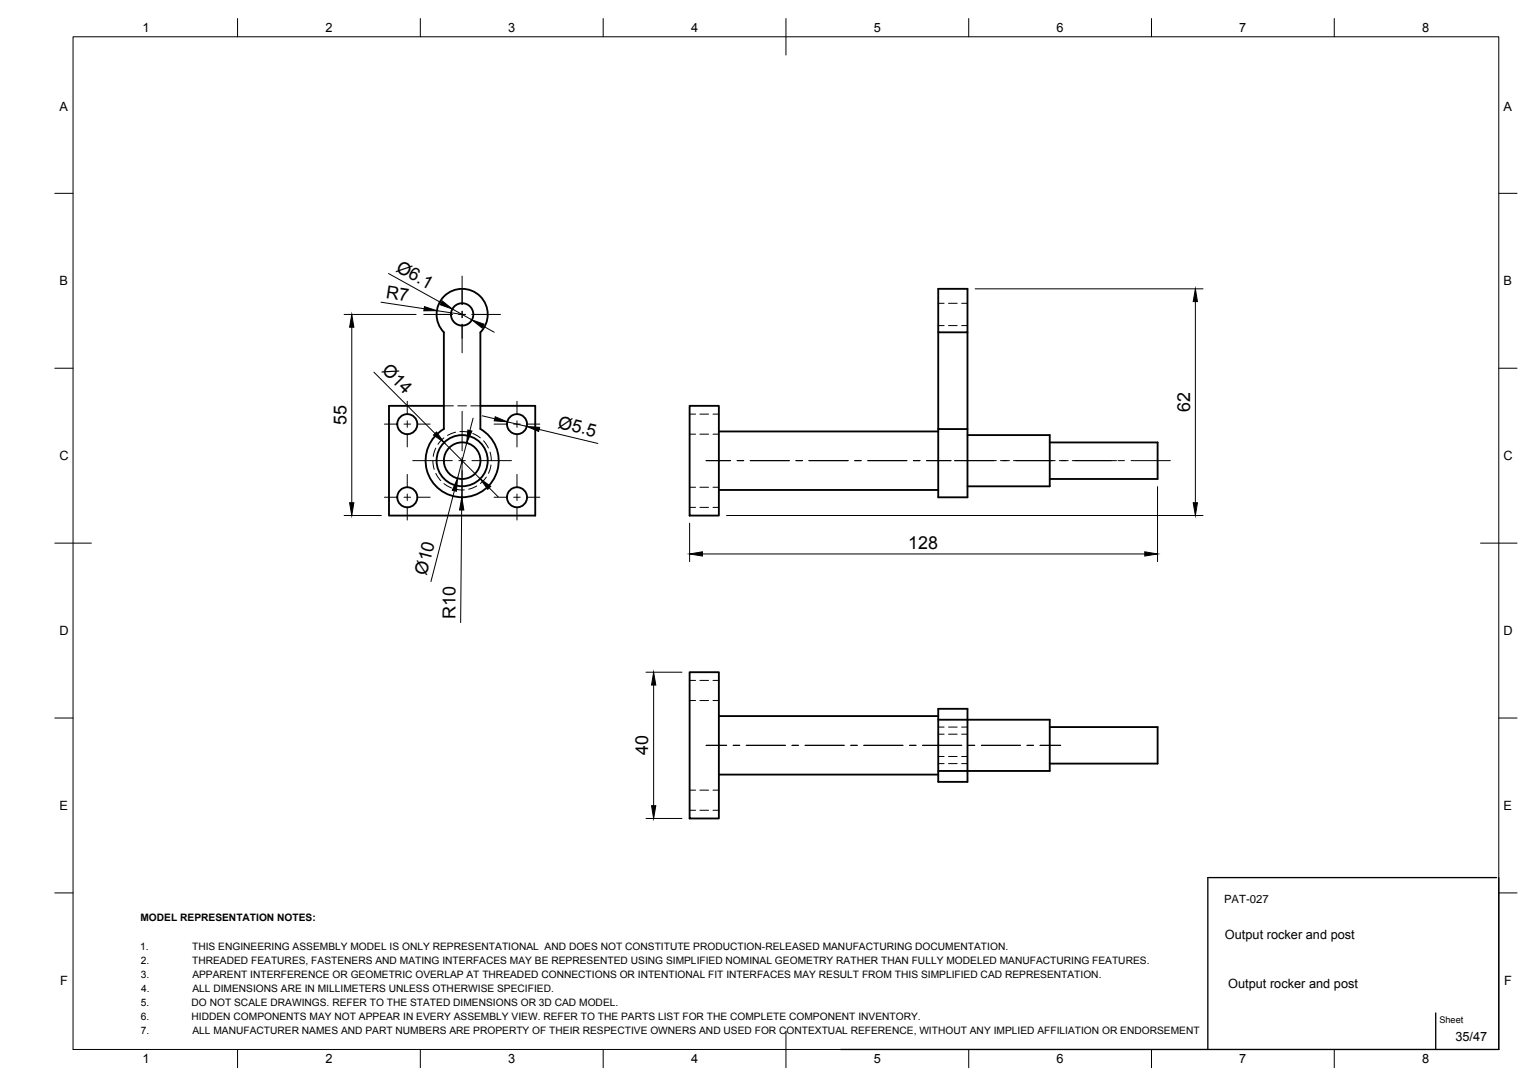
ISO-10303-21;
HEADER;
/* Generated by software containing ST-Developer
 * from STEP Tools, Inc. (www.steptools.com) 
 */

FILE_DESCRIPTION(
/* description */ ('Crank-driven oscillating fan base (mechanism only)'),

/* implementation_level */ '2;1');

FILE_NAME(
/* name */ 'Output rocker and post.step',
/* time_stamp */ '2026-10-28T03:25:00-07:00',
/* author */ (''),
/* organization */ (''),
/* preprocessor_version */ 'ST-DEVELOPER v20.2',
/* originating_system */ 'Autodesk Translation Framework v15.17.0.0',
/* authorisation */ '');

FILE_SCHEMA (('AUTOMOTIVE_DESIGN { 1 0 10303 214 3 1 1 }'));
ENDSEC;

DATA;
#10=MECHANICAL_DESIGN_GEOMETRIC_PRESENTATION_REPRESENTATION('',(#471),#11916);
#383=SHAPE_REPRESENTATION_RELATIONSHIP('SRR','None',#12110,#423);
#423=ADVANCED_BREP_SHAPE_REPRESENTATION('',(#518),#11901);
#471=STYLED_ITEM('',(#12361),#518);
#518=MANIFOLD_SOLID_BREP('Body1',#6102);
#649=FACE_BOUND('',#1640,.T.);
#650=FACE_BOUND('',#1641,.T.);
#651=FACE_BOUND('',#1642,.T.);
#652=FACE_BOUND('',#1643,.T.);
#653=FACE_BOUND('',#1644,.T.);
#654=FACE_BOUND('',#1650,.T.);
#655=FACE_BOUND('',#1651,.T.);
#656=FACE_BOUND('',#1652,.T.);
#657=FACE_BOUND('',#1653,.T.);
#658=FACE_BOUND('',#1659,.T.);
#659=FACE_BOUND('',#1660,.T.);
#660=FACE_BOUND('',#1664,.T.);
#661=FACE_BOUND('',#1665,.T.);
#662=FACE_BOUND('',#1667,.T.);
#815=PLANE('',#7138);
#816=PLANE('',#7140);
#817=PLANE('',#7141);
#818=PLANE('',#7142);
#819=PLANE('',#7143);
#820=PLANE('',#7144);
#821=PLANE('',#7153);
#822=PLANE('',#7154);
#823=PLANE('',#7156);
#824=PLANE('',#7159);
#825=PLANE('',#7161);
#826=PLANE('',#7167);
#1141=FACE_OUTER_BOUND('',#1635,.T.);
#1142=FACE_OUTER_BOUND('',#1636,.T.);
#1143=FACE_OUTER_BOUND('',#1637,.T.);
#1144=FACE_OUTER_BOUND('',#1638,.T.);
#1145=FACE_OUTER_BOUND('',#1639,.T.);
#1146=FACE_OUTER_BOUND('',#1645,.T.);
#1147=FACE_OUTER_BOUND('',#1646,.T.);
#1148=FACE_OUTER_BOUND('',#1647,.T.);
#1149=FACE_OUTER_BOUND('',#1648,.T.);
#1150=FACE_OUTER_BOUND('',#1649,.T.);
#1151=FACE_OUTER_BOUND('',#1654,.T.);
#1152=FACE_OUTER_BOUND('',#1655,.T.);
#1153=FACE_OUTER_BOUND('',#1656,.T.);
#1154=FACE_OUTER_BOUND('',#1657,.T.);
#1155=FACE_OUTER_BOUND('',#1658,.T.);
#1156=FACE_OUTER_BOUND('',#1661,.T.);
#1157=FACE_OUTER_BOUND('',#1662,.T.);
#1158=FACE_OUTER_BOUND('',#1663,.T.);
#1159=FACE_OUTER_BOUND('',#1666,.T.);
#1160=FACE_OUTER_BOUND('',#1668,.T.);
#1161=FACE_OUTER_BOUND('',#1669,.T.);
#1162=FACE_OUTER_BOUND('',#1670,.T.);
#1635=EDGE_LOOP('',(#5098,#5099,#5100,#5101));
#1636=EDGE_LOOP('',(#5102,#5103,#5104,#5105));
#1637=EDGE_LOOP('',(#5106,#5107,#5108,#5109));
#1638=EDGE_LOOP('',(#5110,#5111,#5112,#5113));
#1639=EDGE_LOOP('',(#5114,#5115,#5116,#5117));
#1640=EDGE_LOOP('',(#5118));
#1641=EDGE_LOOP('',(#5119));
#1642=EDGE_LOOP('',(#5120));
#1643=EDGE_LOOP('',(#5121));
#1644=EDGE_LOOP('',(#5122));
#1645=EDGE_LOOP('',(#5123,#5124,#5125,#5126));
#1646=EDGE_LOOP('',(#5127,#5128,#5129,#5130));
#1647=EDGE_LOOP('',(#5131,#5132,#5133,#5134));
#1648=EDGE_LOOP('',(#5135,#5136,#5137,#5138));
#1649=EDGE_LOOP('',(#5139,#5140,#5141,#5142));
#1650=EDGE_LOOP('',(#5143));
#1651=EDGE_LOOP('',(#5144));
#1652=EDGE_LOOP('',(#5145));
#1653=EDGE_LOOP('',(#5146));
#1654=EDGE_LOOP('',(#5147,#5148,#5149,#5150));
#1655=EDGE_LOOP('',(#5151,#5152,#5153,#5154));
#1656=EDGE_LOOP('',(#5155,#5156,#5157,#5158));
#1657=EDGE_LOOP('',(#5159,#5160,#5161,#5162));
#1658=EDGE_LOOP('',(#5163,#5164,#5165,#5166));
#1659=EDGE_LOOP('',(#5167));
#1660=EDGE_LOOP('',(#5168));
#1661=EDGE_LOOP('',(#5169,#5170,#5171,#5172));
#1662=EDGE_LOOP('',(#5173,#5174,#5175,#5176));
#1663=EDGE_LOOP('',(#5177,#5178,#5179,#5180));
#1664=EDGE_LOOP('',(#5181));
#1665=EDGE_LOOP('',(#5182));
#1666=EDGE_LOOP('',(#5183));
#1667=EDGE_LOOP('',(#5184));
#1668=EDGE_LOOP('',(#5185,#5186,#5187,#5188));
#1669=EDGE_LOOP('',(#5189,#5190,#5191,#5192));
#1670=EDGE_LOOP('',(#5193));
#2002=LINE('',#11200,#2335);
#2003=LINE('',#11206,#2336);
#2004=LINE('',#11212,#2337);
#2005=LINE('',#11218,#2338);
#2006=LINE('',#11223,#2339);
#2007=LINE('',#11225,#2340);
#2008=LINE('',#11227,#2341);
#2009=LINE('',#11228,#2342);
#2010=LINE('',#11233,#2343);
#2011=LINE('',#11235,#2344);
#2012=LINE('',#11236,#2345);
#2013=LINE('',#11239,#2346);
#2014=LINE('',#11240,#2347);
#2015=LINE('',#11243,#2348);
#2016=LINE('',#11244,#2349);
#2017=LINE('',#11246,#2350);
#2018=LINE('',#11250,#2351);
#2019=LINE('',#11256,#2352);
#2020=LINE('',#11261,#2353);
#2021=LINE('',#11265,#2354);
#2022=LINE('',#11269,#2355);
#2023=LINE('',#11271,#2356);
#2024=LINE('',#11272,#2357);
#2025=LINE('',#11275,#2358);
#2026=LINE('',#11279,#2359);
#2027=LINE('',#11280,#2360);
#2028=LINE('',#11292,#2361);
#2029=LINE('',#11295,#2362);
#2335=VECTOR('',#8753,0.275);
#2336=VECTOR('',#8760,0.275);
#2337=VECTOR('',#8767,0.275);
#2338=VECTOR('',#8774,0.275);
#2339=VECTOR('',#8779,1.);
#2340=VECTOR('',#8780,1.);
#2341=VECTOR('',#8781,1.);
#2342=VECTOR('',#8782,1.);
#2343=VECTOR('',#8787,1.);
#2344=VECTOR('',#8788,1.);
#2345=VECTOR('',#8789,1.);
#2346=VECTOR('',#8792,1.);
#2347=VECTOR('',#8793,1.);
#2348=VECTOR('',#8796,1.);
#2349=VECTOR('',#8797,1.);
#2350=VECTOR('',#8800,1.);
#2351=VECTOR('',#8805,0.800000000000001);
#2352=VECTOR('',#8812,0.305);
#2353=VECTOR('',#8817,1.);
#2354=VECTOR('',#8820,1.);
#2355=VECTOR('',#8825,1.);
#2356=VECTOR('',#8826,1.);
#2357=VECTOR('',#8827,1.);
#2358=VECTOR('',#8830,1.);
#2359=VECTOR('',#8835,1.);
#2360=VECTOR('',#8836,1.);
#2361=VECTOR('',#8853,0.699999999999999);
#2362=VECTOR('',#8856,0.5);
#2739=CIRCLE('',#7127,0.275);
#2740=CIRCLE('',#7128,0.275);
#2741=CIRCLE('',#7130,0.275);
#2742=CIRCLE('',#7131,0.275);
#2743=CIRCLE('',#7133,0.275);
#2744=CIRCLE('',#7134,0.275);
#2745=CIRCLE('',#7136,0.275);
#2746=CIRCLE('',#7137,0.275);
#2747=CIRCLE('',#7139,0.800000000000001);
#2748=CIRCLE('',#7146,0.800000000000001);
#2749=CIRCLE('',#7148,0.305);
#2750=CIRCLE('',#7149,0.305);
#2751=CIRCLE('',#7151,0.699999999999999);
#2752=CIRCLE('',#7152,0.699999999999999);
#2753=CIRCLE('',#7155,1.);
#2754=CIRCLE('',#7158,1.);
#2755=CIRCLE('',#7160,0.699999999999999);
#2756=CIRCLE('',#7162,0.699999999999999);
#2757=CIRCLE('',#7163,0.5);
#2758=CIRCLE('',#7166,0.5);
#3182=VERTEX_POINT('',#11197);
#3183=VERTEX_POINT('',#11199);
#3184=VERTEX_POINT('',#11203);
#3185=VERTEX_POINT('',#11205);
#3186=VERTEX_POINT('',#11209);
#3187=VERTEX_POINT('',#11211);
#3188=VERTEX_POINT('',#11215);
#3189=VERTEX_POINT('',#11217);
#3190=VERTEX_POINT('',#11221);
#3191=VERTEX_POINT('',#11222);
#3192=VERTEX_POINT('',#11224);
#3193=VERTEX_POINT('',#11226);
#3194=VERTEX_POINT('',#11229);
#3195=VERTEX_POINT('',#11232);
#3196=VERTEX_POINT('',#11234);
#3197=VERTEX_POINT('',#11238);
#3198=VERTEX_POINT('',#11242);
#3199=VERTEX_POINT('',#11249);
#3200=VERTEX_POINT('',#11253);
#3201=VERTEX_POINT('',#11255);
#3202=VERTEX_POINT('',#11259);
#3203=VERTEX_POINT('',#11260);
#3204=VERTEX_POINT('',#11262);
#3205=VERTEX_POINT('',#11264);
#3206=VERTEX_POINT('',#11268);
#3207=VERTEX_POINT('',#11270);
#3208=VERTEX_POINT('',#11274);
#3209=VERTEX_POINT('',#11278);
#3210=VERTEX_POINT('',#11284);
#3211=VERTEX_POINT('',#11287);
#3212=VERTEX_POINT('',#11289);
#3213=VERTEX_POINT('',#11294);
#3844=EDGE_CURVE('',#3182,#3182,#2739,.T.);
#3845=EDGE_CURVE('',#3182,#3183,#2002,.T.);
#3846=EDGE_CURVE('',#3183,#3183,#2740,.T.);
#3847=EDGE_CURVE('',#3184,#3184,#2741,.T.);
#3848=EDGE_CURVE('',#3184,#3185,#2003,.T.);
#3849=EDGE_CURVE('',#3185,#3185,#2742,.T.);
#3850=EDGE_CURVE('',#3186,#3186,#2743,.T.);
#3851=EDGE_CURVE('',#3186,#3187,#2004,.T.);
#3852=EDGE_CURVE('',#3187,#3187,#2744,.T.);
#3853=EDGE_CURVE('',#3188,#3188,#2745,.T.);
#3854=EDGE_CURVE('',#3188,#3189,#2005,.T.);
#3855=EDGE_CURVE('',#3189,#3189,#2746,.T.);
#3856=EDGE_CURVE('',#3190,#3191,#2006,.T.);
#3857=EDGE_CURVE('',#3192,#3190,#2007,.T.);
#3858=EDGE_CURVE('',#3193,#3192,#2008,.T.);
#3859=EDGE_CURVE('',#3191,#3193,#2009,.T.);
#3860=EDGE_CURVE('',#3194,#3194,#2747,.T.);
#3861=EDGE_CURVE('',#3190,#3195,#2010,.T.);
#3862=EDGE_CURVE('',#3196,#3195,#2011,.T.);
#3863=EDGE_CURVE('',#3192,#3196,#2012,.T.);
#3864=EDGE_CURVE('',#3197,#3196,#2013,.T.);
#3865=EDGE_CURVE('',#3193,#3197,#2014,.T.);
#3866=EDGE_CURVE('',#3198,#3197,#2015,.T.);
#3867=EDGE_CURVE('',#3191,#3198,#2016,.T.);
#3868=EDGE_CURVE('',#3195,#3198,#2017,.T.);
#3869=EDGE_CURVE('',#3194,#3199,#2018,.T.);
#3870=EDGE_CURVE('',#3199,#3199,#2748,.T.);
#3871=EDGE_CURVE('',#3200,#3200,#2749,.T.);
#3872=EDGE_CURVE('',#3200,#3201,#2019,.T.);
#3873=EDGE_CURVE('',#3201,#3201,#2750,.T.);
#3874=EDGE_CURVE('',#3202,#3203,#2020,.T.);
#3875=EDGE_CURVE('',#3202,#3204,#2751,.T.);
#3876=EDGE_CURVE('',#3205,#3204,#2021,.T.);
#3877=EDGE_CURVE('',#3203,#3205,#2752,.T.);
#3878=EDGE_CURVE('',#3206,#3203,#2022,.T.);
#3879=EDGE_CURVE('',#3207,#3206,#2023,.T.);
#3880=EDGE_CURVE('',#3202,#3207,#2024,.T.);
#3881=EDGE_CURVE('',#3205,#3208,#2025,.T.);
#3882=EDGE_CURVE('',#3208,#3206,#2753,.T.);
#3883=EDGE_CURVE('',#3209,#3204,#2026,.T.);
#3884=EDGE_CURVE('',#3208,#3209,#2027,.T.);
#3885=EDGE_CURVE('',#3209,#3207,#2754,.T.);
#3886=EDGE_CURVE('',#3210,#3210,#2755,.T.);
#3887=EDGE_CURVE('',#3211,#3211,#2756,.T.);
#3888=EDGE_CURVE('',#3212,#3212,#2757,.T.);
#3889=EDGE_CURVE('',#3210,#3211,#2028,.T.);
#3890=EDGE_CURVE('',#3212,#3213,#2029,.T.);
#3891=EDGE_CURVE('',#3213,#3213,#2758,.T.);
#5098=ORIENTED_EDGE('',*,*,#3844,.F.);
#5099=ORIENTED_EDGE('',*,*,#3845,.T.);
#5100=ORIENTED_EDGE('',*,*,#3846,.F.);
#5101=ORIENTED_EDGE('',*,*,#3845,.F.);
#5102=ORIENTED_EDGE('',*,*,#3847,.F.);
#5103=ORIENTED_EDGE('',*,*,#3848,.T.);
#5104=ORIENTED_EDGE('',*,*,#3849,.F.);
#5105=ORIENTED_EDGE('',*,*,#3848,.F.);
#5106=ORIENTED_EDGE('',*,*,#3850,.F.);
#5107=ORIENTED_EDGE('',*,*,#3851,.T.);
#5108=ORIENTED_EDGE('',*,*,#3852,.F.);
#5109=ORIENTED_EDGE('',*,*,#3851,.F.);
#5110=ORIENTED_EDGE('',*,*,#3853,.F.);
#5111=ORIENTED_EDGE('',*,*,#3854,.T.);
#5112=ORIENTED_EDGE('',*,*,#3855,.F.);
#5113=ORIENTED_EDGE('',*,*,#3854,.F.);
#5114=ORIENTED_EDGE('',*,*,#3856,.F.);
#5115=ORIENTED_EDGE('',*,*,#3857,.F.);
#5116=ORIENTED_EDGE('',*,*,#3858,.F.);
#5117=ORIENTED_EDGE('',*,*,#3859,.F.);
#5118=ORIENTED_EDGE('',*,*,#3860,.T.);
#5119=ORIENTED_EDGE('',*,*,#3853,.T.);
#5120=ORIENTED_EDGE('',*,*,#3850,.T.);
#5121=ORIENTED_EDGE('',*,*,#3847,.T.);
#5122=ORIENTED_EDGE('',*,*,#3844,.T.);
#5123=ORIENTED_EDGE('',*,*,#3857,.T.);
#5124=ORIENTED_EDGE('',*,*,#3861,.T.);
#5125=ORIENTED_EDGE('',*,*,#3862,.F.);
#5126=ORIENTED_EDGE('',*,*,#3863,.F.);
#5127=ORIENTED_EDGE('',*,*,#3858,.T.);
#5128=ORIENTED_EDGE('',*,*,#3863,.T.);
#5129=ORIENTED_EDGE('',*,*,#3864,.F.);
#5130=ORIENTED_EDGE('',*,*,#3865,.F.);
#5131=ORIENTED_EDGE('',*,*,#3859,.T.);
#5132=ORIENTED_EDGE('',*,*,#3865,.T.);
#5133=ORIENTED_EDGE('',*,*,#3866,.F.);
#5134=ORIENTED_EDGE('',*,*,#3867,.F.);
#5135=ORIENTED_EDGE('',*,*,#3856,.T.);
#5136=ORIENTED_EDGE('',*,*,#3867,.T.);
#5137=ORIENTED_EDGE('',*,*,#3868,.F.);
#5138=ORIENTED_EDGE('',*,*,#3861,.F.);
#5139=ORIENTED_EDGE('',*,*,#3868,.T.);
#5140=ORIENTED_EDGE('',*,*,#3866,.T.);
#5141=ORIENTED_EDGE('',*,*,#3864,.T.);
#5142=ORIENTED_EDGE('',*,*,#3862,.T.);
#5143=ORIENTED_EDGE('',*,*,#3846,.T.);
#5144=ORIENTED_EDGE('',*,*,#3849,.T.);
#5145=ORIENTED_EDGE('',*,*,#3852,.T.);
#5146=ORIENTED_EDGE('',*,*,#3855,.T.);
#5147=ORIENTED_EDGE('',*,*,#3860,.F.);
#5148=ORIENTED_EDGE('',*,*,#3869,.T.);
#5149=ORIENTED_EDGE('',*,*,#3870,.F.);
#5150=ORIENTED_EDGE('',*,*,#3869,.F.);
#5151=ORIENTED_EDGE('',*,*,#3871,.F.);
#5152=ORIENTED_EDGE('',*,*,#3872,.T.);
#5153=ORIENTED_EDGE('',*,*,#3873,.F.);
#5154=ORIENTED_EDGE('',*,*,#3872,.F.);
#5155=ORIENTED_EDGE('',*,*,#3874,.F.);
#5156=ORIENTED_EDGE('',*,*,#3875,.T.);
#5157=ORIENTED_EDGE('',*,*,#3876,.F.);
#5158=ORIENTED_EDGE('',*,*,#3877,.F.);
#5159=ORIENTED_EDGE('',*,*,#3874,.T.);
#5160=ORIENTED_EDGE('',*,*,#3878,.F.);
#5161=ORIENTED_EDGE('',*,*,#3879,.F.);
#5162=ORIENTED_EDGE('',*,*,#3880,.F.);
#5163=ORIENTED_EDGE('',*,*,#3877,.T.);
#5164=ORIENTED_EDGE('',*,*,#3881,.T.);
#5165=ORIENTED_EDGE('',*,*,#3882,.T.);
#5166=ORIENTED_EDGE('',*,*,#3878,.T.);
#5167=ORIENTED_EDGE('',*,*,#3870,.T.);
#5168=ORIENTED_EDGE('',*,*,#3873,.T.);
#5169=ORIENTED_EDGE('',*,*,#3876,.T.);
#5170=ORIENTED_EDGE('',*,*,#3883,.F.);
#5171=ORIENTED_EDGE('',*,*,#3884,.F.);
#5172=ORIENTED_EDGE('',*,*,#3881,.F.);
#5173=ORIENTED_EDGE('',*,*,#3884,.T.);
#5174=ORIENTED_EDGE('',*,*,#3885,.T.);
#5175=ORIENTED_EDGE('',*,*,#3879,.T.);
#5176=ORIENTED_EDGE('',*,*,#3882,.F.);
#5177=ORIENTED_EDGE('',*,*,#3880,.T.);
#5178=ORIENTED_EDGE('',*,*,#3885,.F.);
#5179=ORIENTED_EDGE('',*,*,#3883,.T.);
#5180=ORIENTED_EDGE('',*,*,#3875,.F.);
#5181=ORIENTED_EDGE('',*,*,#3871,.T.);
#5182=ORIENTED_EDGE('',*,*,#3886,.T.);
#5183=ORIENTED_EDGE('',*,*,#3887,.F.);
#5184=ORIENTED_EDGE('',*,*,#3888,.F.);
#5185=ORIENTED_EDGE('',*,*,#3886,.F.);
#5186=ORIENTED_EDGE('',*,*,#3889,.T.);
#5187=ORIENTED_EDGE('',*,*,#3887,.T.);
#5188=ORIENTED_EDGE('',*,*,#3889,.F.);
#5189=ORIENTED_EDGE('',*,*,#3888,.T.);
#5190=ORIENTED_EDGE('',*,*,#3890,.T.);
#5191=ORIENTED_EDGE('',*,*,#3891,.T.);
#5192=ORIENTED_EDGE('',*,*,#3890,.F.);
#5193=ORIENTED_EDGE('',*,*,#3891,.F.);
#5651=CYLINDRICAL_SURFACE('',#7126,0.275);
#5652=CYLINDRICAL_SURFACE('',#7129,0.275);
#5653=CYLINDRICAL_SURFACE('',#7132,0.275);
#5654=CYLINDRICAL_SURFACE('',#7135,0.275);
#5655=CYLINDRICAL_SURFACE('',#7145,0.800000000000001);
#5656=CYLINDRICAL_SURFACE('',#7147,0.305);
#5657=CYLINDRICAL_SURFACE('',#7150,0.699999999999999);
#5658=CYLINDRICAL_SURFACE('',#7157,1.);
#5659=CYLINDRICAL_SURFACE('',#7164,0.699999999999999);
#5660=CYLINDRICAL_SURFACE('',#7165,0.5);
#5947=ADVANCED_FACE('',(#1141),#5651,.F.);
#5948=ADVANCED_FACE('',(#1142),#5652,.F.);
#5949=ADVANCED_FACE('',(#1143),#5653,.F.);
#5950=ADVANCED_FACE('',(#1144),#5654,.F.);
#5951=ADVANCED_FACE('',(#1145,#649,#650,#651,#652,#653),#815,.F.);
#5952=ADVANCED_FACE('',(#1146),#816,.T.);
#5953=ADVANCED_FACE('',(#1147),#817,.T.);
#5954=ADVANCED_FACE('',(#1148),#818,.T.);
#5955=ADVANCED_FACE('',(#1149),#819,.T.);
#5956=ADVANCED_FACE('',(#1150,#654,#655,#656,#657),#820,.T.);
#5957=ADVANCED_FACE('',(#1151),#5655,.T.);
#5958=ADVANCED_FACE('',(#1152),#5656,.F.);
#5959=ADVANCED_FACE('',(#1153),#5657,.T.);
#5960=ADVANCED_FACE('',(#1154),#821,.T.);
#5961=ADVANCED_FACE('',(#1155,#658,#659),#822,.T.);
#5962=ADVANCED_FACE('',(#1156),#823,.T.);
#5963=ADVANCED_FACE('',(#1157),#5658,.T.);
#5964=ADVANCED_FACE('',(#1158,#660,#661),#824,.F.);
#5965=ADVANCED_FACE('',(#1159,#662),#825,.F.);
#5966=ADVANCED_FACE('',(#1160),#5659,.T.);
#5967=ADVANCED_FACE('',(#1161),#5660,.T.);
#5968=ADVANCED_FACE('',(#1162),#826,.F.);
#6102=CLOSED_SHELL('',(#5947,#5948,#5949,#5950,#5951,#5952,#5953,#5954,
#5955,#5956,#5957,#5958,#5959,#5960,#5961,#5962,#5963,#5964,#5965,#5966,
#5967,#5968));
#7125=AXIS2_PLACEMENT_3D('',#11195,#8747,#8748);
#7126=AXIS2_PLACEMENT_3D('',#11196,#8749,#8750);
#7127=AXIS2_PLACEMENT_3D('',#11198,#8751,#8752);
#7128=AXIS2_PLACEMENT_3D('',#11201,#8754,#8755);
#7129=AXIS2_PLACEMENT_3D('',#11202,#8756,#8757);
#7130=AXIS2_PLACEMENT_3D('',#11204,#8758,#8759);
#7131=AXIS2_PLACEMENT_3D('',#11207,#8761,#8762);
#7132=AXIS2_PLACEMENT_3D('',#11208,#8763,#8764);
#7133=AXIS2_PLACEMENT_3D('',#11210,#8765,#8766);
#7134=AXIS2_PLACEMENT_3D('',#11213,#8768,#8769);
#7135=AXIS2_PLACEMENT_3D('',#11214,#8770,#8771);
#7136=AXIS2_PLACEMENT_3D('',#11216,#8772,#8773);
#7137=AXIS2_PLACEMENT_3D('',#11219,#8775,#8776);
#7138=AXIS2_PLACEMENT_3D('',#11220,#8777,#8778);
#7139=AXIS2_PLACEMENT_3D('',#11230,#8783,#8784);
#7140=AXIS2_PLACEMENT_3D('',#11231,#8785,#8786);
#7141=AXIS2_PLACEMENT_3D('',#11237,#8790,#8791);
#7142=AXIS2_PLACEMENT_3D('',#11241,#8794,#8795);
#7143=AXIS2_PLACEMENT_3D('',#11245,#8798,#8799);
#7144=AXIS2_PLACEMENT_3D('',#11247,#8801,#8802);
#7145=AXIS2_PLACEMENT_3D('',#11248,#8803,#8804);
#7146=AXIS2_PLACEMENT_3D('',#11251,#8806,#8807);
#7147=AXIS2_PLACEMENT_3D('',#11252,#8808,#8809);
#7148=AXIS2_PLACEMENT_3D('',#11254,#8810,#8811);
#7149=AXIS2_PLACEMENT_3D('',#11257,#8813,#8814);
#7150=AXIS2_PLACEMENT_3D('',#11258,#8815,#8816);
#7151=AXIS2_PLACEMENT_3D('',#11263,#8818,#8819);
#7152=AXIS2_PLACEMENT_3D('',#11266,#8821,#8822);
#7153=AXIS2_PLACEMENT_3D('',#11267,#8823,#8824);
#7154=AXIS2_PLACEMENT_3D('',#11273,#8828,#8829);
#7155=AXIS2_PLACEMENT_3D('',#11276,#8831,#8832);
#7156=AXIS2_PLACEMENT_3D('',#11277,#8833,#8834);
#7157=AXIS2_PLACEMENT_3D('',#11281,#8837,#8838);
#7158=AXIS2_PLACEMENT_3D('',#11282,#8839,#8840);
#7159=AXIS2_PLACEMENT_3D('',#11283,#8841,#8842);
#7160=AXIS2_PLACEMENT_3D('',#11285,#8843,#8844);
#7161=AXIS2_PLACEMENT_3D('',#11286,#8845,#8846);
#7162=AXIS2_PLACEMENT_3D('',#11288,#8847,#8848);
#7163=AXIS2_PLACEMENT_3D('',#11290,#8849,#8850);
#7164=AXIS2_PLACEMENT_3D('',#11291,#8851,#8852);
#7165=AXIS2_PLACEMENT_3D('',#11293,#8854,#8855);
#7166=AXIS2_PLACEMENT_3D('',#11296,#8857,#8858);
#7167=AXIS2_PLACEMENT_3D('',#11297,#8859,#8860);
#8747=DIRECTION('axis',(0.,0.,1.));
#8748=DIRECTION('refdir',(1.,0.,0.));
#8749=DIRECTION('center_axis',(0.,0.,1.));
#8750=DIRECTION('ref_axis',(1.,0.,0.));
#8751=DIRECTION('center_axis',(0.,0.,1.));
#8752=DIRECTION('ref_axis',(1.,0.,0.));
#8753=DIRECTION('',(0.,0.,1.));
#8754=DIRECTION('center_axis',(0.,0.,-1.));
#8755=DIRECTION('ref_axis',(1.,0.,0.));
#8756=DIRECTION('center_axis',(0.,0.,1.));
#8757=DIRECTION('ref_axis',(1.,0.,0.));
#8758=DIRECTION('center_axis',(0.,0.,1.));
#8759=DIRECTION('ref_axis',(1.,0.,0.));
#8760=DIRECTION('',(0.,0.,1.));
#8761=DIRECTION('center_axis',(0.,0.,-1.));
#8762=DIRECTION('ref_axis',(1.,0.,0.));
#8763=DIRECTION('center_axis',(0.,0.,1.));
#8764=DIRECTION('ref_axis',(1.,0.,0.));
#8765=DIRECTION('center_axis',(0.,0.,1.));
#8766=DIRECTION('ref_axis',(1.,0.,0.));
#8767=DIRECTION('',(0.,0.,1.));
#8768=DIRECTION('center_axis',(0.,0.,-1.));
#8769=DIRECTION('ref_axis',(1.,0.,0.));
#8770=DIRECTION('center_axis',(0.,0.,1.));
#8771=DIRECTION('ref_axis',(1.,0.,0.));
#8772=DIRECTION('center_axis',(0.,0.,1.));
#8773=DIRECTION('ref_axis',(1.,0.,0.));
#8774=DIRECTION('',(0.,0.,1.));
#8775=DIRECTION('center_axis',(0.,0.,-1.));
#8776=DIRECTION('ref_axis',(1.,0.,0.));
#8777=DIRECTION('center_axis',(0.,0.,1.));
#8778=DIRECTION('ref_axis',(1.,0.,0.));
#8779=DIRECTION('',(0.,-1.,0.));
#8780=DIRECTION('',(-1.,0.,0.));
#8781=DIRECTION('',(0.,1.,0.));
#8782=DIRECTION('',(1.,0.,0.));
#8783=DIRECTION('center_axis',(0.,0.,1.));
#8784=DIRECTION('ref_axis',(1.,0.,0.));
#8785=DIRECTION('center_axis',(0.,1.,0.));
#8786=DIRECTION('ref_axis',(-1.,0.,0.));
#8787=DIRECTION('',(0.,0.,1.));
#8788=DIRECTION('',(-1.,0.,0.));
#8789=DIRECTION('',(0.,0.,1.));
#8790=DIRECTION('center_axis',(1.,0.,0.));
#8791=DIRECTION('ref_axis',(0.,1.,0.));
#8792=DIRECTION('',(0.,1.,0.));
#8793=DIRECTION('',(0.,0.,1.));
#8794=DIRECTION('center_axis',(0.,-1.,0.));
#8795=DIRECTION('ref_axis',(1.,0.,0.));
#8796=DIRECTION('',(1.,0.,0.));
#8797=DIRECTION('',(0.,0.,1.));
#8798=DIRECTION('center_axis',(-1.,0.,0.));
#8799=DIRECTION('ref_axis',(0.,-1.,0.));
#8800=DIRECTION('',(0.,-1.,0.));
#8801=DIRECTION('center_axis',(0.,0.,1.));
#8802=DIRECTION('ref_axis',(1.,0.,0.));
#8803=DIRECTION('center_axis',(0.,0.,1.));
#8804=DIRECTION('ref_axis',(1.,0.,0.));
#8805=DIRECTION('',(0.,0.,-1.));
#8806=DIRECTION('center_axis',(0.,0.,-1.));
#8807=DIRECTION('ref_axis',(1.,0.,0.));
#8808=DIRECTION('center_axis',(0.,0.,1.));
#8809=DIRECTION('ref_axis',(1.,0.,0.));
#8810=DIRECTION('center_axis',(0.,0.,1.));
#8811=DIRECTION('ref_axis',(1.,0.,0.));
#8812=DIRECTION('',(0.,0.,1.));
#8813=DIRECTION('center_axis',(0.,0.,-1.));
#8814=DIRECTION('ref_axis',(1.,0.,0.));
#8815=DIRECTION('center_axis',(0.,0.,1.));
#8816=DIRECTION('ref_axis',(6.12323399573677E-17,1.,0.));
#8817=DIRECTION('',(0.,0.,1.));
#8818=DIRECTION('center_axis',(0.,0.,1.));
#8819=DIRECTION('ref_axis',(1.,0.,0.));
#8820=DIRECTION('',(0.,0.,-1.));
#8821=DIRECTION('center_axis',(0.,0.,1.));
#8822=DIRECTION('ref_axis',(1.,0.,0.));
#8823=DIRECTION('center_axis',(1.,0.,0.));
#8824=DIRECTION('ref_axis',(0.,1.,0.));
#8825=DIRECTION('',(0.,1.,0.));
#8826=DIRECTION('',(0.,0.,1.));
#8827=DIRECTION('',(0.,-1.,0.));
#8828=DIRECTION('center_axis',(0.,0.,1.));
#8829=DIRECTION('ref_axis',(1.,0.,0.));
#8830=DIRECTION('',(0.,-1.,0.));
#8831=DIRECTION('center_axis',(0.,0.,1.));
#8832=DIRECTION('ref_axis',(1.,0.,0.));
#8833=DIRECTION('center_axis',(-1.,0.,0.));
#8834=DIRECTION('ref_axis',(0.,-1.,0.));
#8835=DIRECTION('',(0.,1.,0.));
#8836=DIRECTION('',(0.,0.,-1.));
#8837=DIRECTION('center_axis',(0.,0.,1.));
#8838=DIRECTION('ref_axis',(-1.83697019872103E-16,-1.,0.));
#8839=DIRECTION('center_axis',(0.,0.,1.));
#8840=DIRECTION('ref_axis',(1.,0.,0.));
#8841=DIRECTION('center_axis',(0.,0.,1.));
#8842=DIRECTION('ref_axis',(1.,0.,0.));
#8843=DIRECTION('center_axis',(0.,0.,1.));
#8844=DIRECTION('ref_axis',(1.,0.,0.));
#8845=DIRECTION('center_axis',(0.,0.,1.));
#8846=DIRECTION('ref_axis',(1.,0.,0.));
#8847=DIRECTION('center_axis',(0.,0.,1.));
#8848=DIRECTION('ref_axis',(1.,0.,0.));
#8849=DIRECTION('center_axis',(0.,0.,-1.));
#8850=DIRECTION('ref_axis',(1.,0.,0.));
#8851=DIRECTION('center_axis',(0.,0.,1.));
#8852=DIRECTION('ref_axis',(1.,0.,0.));
#8853=DIRECTION('',(0.,0.,-1.));
#8854=DIRECTION('center_axis',(0.,0.,1.));
#8855=DIRECTION('ref_axis',(1.,0.,0.));
#8856=DIRECTION('',(0.,0.,-1.));
#8857=DIRECTION('center_axis',(0.,0.,1.));
#8858=DIRECTION('ref_axis',(1.,0.,0.));
#8859=DIRECTION('center_axis',(0.,0.,1.));
#8860=DIRECTION('ref_axis',(1.,0.,0.));
#11195=CARTESIAN_POINT('',(0.,0.,0.));
#11196=CARTESIAN_POINT('Origin',(9.5,-1.,12.9));
#11197=CARTESIAN_POINT('',(9.225,-1.,13.));
#11198=CARTESIAN_POINT('Origin',(9.5,-1.,13.));
#11199=CARTESIAN_POINT('',(9.225,-1.,13.8));
#11200=CARTESIAN_POINT('',(9.225,-1.,12.9));
#11201=CARTESIAN_POINT('Origin',(9.5,-1.,13.8));
#11202=CARTESIAN_POINT('Origin',(6.5,1.,12.9));
#11203=CARTESIAN_POINT('',(6.225,1.,13.));
#11204=CARTESIAN_POINT('Origin',(6.5,1.,13.));
#11205=CARTESIAN_POINT('',(6.225,1.,13.8));
#11206=CARTESIAN_POINT('',(6.225,1.,12.9));
#11207=CARTESIAN_POINT('Origin',(6.5,1.,13.8));
#11208=CARTESIAN_POINT('Origin',(6.5,-1.,12.9));
#11209=CARTESIAN_POINT('',(6.225,-1.,13.));
#11210=CARTESIAN_POINT('Origin',(6.5,-1.,13.));
#11211=CARTESIAN_POINT('',(6.225,-1.,13.8));
#11212=CARTESIAN_POINT('',(6.225,-1.,12.9));
#11213=CARTESIAN_POINT('Origin',(6.5,-1.,13.8));
#11214=CARTESIAN_POINT('Origin',(9.5,1.,12.9));
#11215=CARTESIAN_POINT('',(9.225,1.,13.));
#11216=CARTESIAN_POINT('Origin',(9.5,1.,13.));
#11217=CARTESIAN_POINT('',(9.225,1.,13.8));
#11218=CARTESIAN_POINT('',(9.225,1.,12.9));
#11219=CARTESIAN_POINT('Origin',(9.5,1.,13.8));
#11220=CARTESIAN_POINT('Origin',(8.,0.,13.));
#11221=CARTESIAN_POINT('',(6.,1.5,13.));
#11222=CARTESIAN_POINT('',(6.,-1.5,13.));
#11223=CARTESIAN_POINT('',(6.,1.5,13.));
#11224=CARTESIAN_POINT('',(10.,1.5,13.));
#11225=CARTESIAN_POINT('',(10.,1.5,13.));
#11226=CARTESIAN_POINT('',(10.,-1.5,13.));
#11227=CARTESIAN_POINT('',(10.,-1.5,13.));
#11228=CARTESIAN_POINT('',(6.,-1.5,13.));
#11229=CARTESIAN_POINT('',(7.2,-9.79717439317883E-17,13.));
#11230=CARTESIAN_POINT('Origin',(8.,0.,13.));
#11231=CARTESIAN_POINT('Origin',(10.,1.5,13.));
#11232=CARTESIAN_POINT('',(6.,1.5,13.8));
#11233=CARTESIAN_POINT('',(6.,1.5,13.));
#11234=CARTESIAN_POINT('',(10.,1.5,13.8));
#11235=CARTESIAN_POINT('',(10.,1.5,13.8));
#11236=CARTESIAN_POINT('',(10.,1.5,13.));
#11237=CARTESIAN_POINT('Origin',(10.,-1.5,13.));
#11238=CARTESIAN_POINT('',(10.,-1.5,13.8));
#11239=CARTESIAN_POINT('',(10.,-1.5,13.8));
#11240=CARTESIAN_POINT('',(10.,-1.5,13.));
#11241=CARTESIAN_POINT('Origin',(6.,-1.5,13.));
#11242=CARTESIAN_POINT('',(6.,-1.5,13.8));
#11243=CARTESIAN_POINT('',(6.,-1.5,13.8));
#11244=CARTESIAN_POINT('',(6.,-1.5,13.));
#11245=CARTESIAN_POINT('Origin',(6.,1.5,13.));
#11246=CARTESIAN_POINT('',(6.,1.5,13.8));
#11247=CARTESIAN_POINT('Origin',(8.,0.,13.8));
#11248=CARTESIAN_POINT('Origin',(8.,0.,7.));
#11249=CARTESIAN_POINT('',(7.2,-9.79717439317883E-17,7.));
#11250=CARTESIAN_POINT('',(7.2,-9.79717439317883E-17,7.));
#11251=CARTESIAN_POINT('Origin',(8.,0.,7.));
#11252=CARTESIAN_POINT('Origin',(8.,4.,6.1));
#11253=CARTESIAN_POINT('',(7.695,4.,6.2));
#11254=CARTESIAN_POINT('Origin',(8.,4.,6.2));
#11255=CARTESIAN_POINT('',(7.695,4.,7.));
#11256=CARTESIAN_POINT('',(7.695,4.,6.1));
#11257=CARTESIAN_POINT('Origin',(8.,4.,7.));
#11258=CARTESIAN_POINT('Origin',(8.,4.,6.2));
#11259=CARTESIAN_POINT('',(8.5,3.51010205144337,6.2));
#11260=CARTESIAN_POINT('',(8.5,3.51010205144337,7.));
#11261=CARTESIAN_POINT('',(8.5,3.51010205144337,6.2));
#11262=CARTESIAN_POINT('',(7.5,3.51010205144337,6.2));
#11263=CARTESIAN_POINT('Origin',(8.,4.,6.2));
#11264=CARTESIAN_POINT('',(7.5,3.51010205144337,7.));
#11265=CARTESIAN_POINT('',(7.5,3.51010205144337,6.2));
#11266=CARTESIAN_POINT('Origin',(8.,4.,7.));
#11267=CARTESIAN_POINT('Origin',(8.5,0.,6.2));
#11268=CARTESIAN_POINT('',(8.5,0.866025403784439,7.));
#11269=CARTESIAN_POINT('',(8.5,4.,7.));
#11270=CARTESIAN_POINT('',(8.5,0.866025403784439,6.2));
#11271=CARTESIAN_POINT('',(8.5,0.866025403784439,6.2));
#11272=CARTESIAN_POINT('',(8.5,4.,6.2));
#11273=CARTESIAN_POINT('Origin',(8.,0.,7.));
#11274=CARTESIAN_POINT('',(7.5,0.866025403784439,7.));
#11275=CARTESIAN_POINT('',(7.5,0.,7.));
#11276=CARTESIAN_POINT('Origin',(8.,0.,7.));
#11277=CARTESIAN_POINT('Origin',(7.5,4.,6.2));
#11278=CARTESIAN_POINT('',(7.5,0.866025403784439,6.2));
#11279=CARTESIAN_POINT('',(7.5,0.,6.2));
#11280=CARTESIAN_POINT('',(7.5,0.866025403784439,6.2));
#11281=CARTESIAN_POINT('Origin',(8.,0.,6.2));
#11282=CARTESIAN_POINT('Origin',(8.,0.,6.2));
#11283=CARTESIAN_POINT('Origin',(8.,0.,6.2));
#11284=CARTESIAN_POINT('',(7.3,-8.57252759403146E-17,6.2));
#11285=CARTESIAN_POINT('Origin',(8.,0.,6.2));
#11286=CARTESIAN_POINT('Origin',(8.,0.,3.95));
#11287=CARTESIAN_POINT('',(7.3,-8.57252759403146E-17,3.95));
#11288=CARTESIAN_POINT('Origin',(8.,0.,3.95));
#11289=CARTESIAN_POINT('',(7.5,6.12323399573677E-17,3.95));
#11290=CARTESIAN_POINT('Origin',(8.,0.,3.95));
#11291=CARTESIAN_POINT('Origin',(8.,0.,3.95));
#11292=CARTESIAN_POINT('',(7.3,-8.57252759403146E-17,3.95));
#11293=CARTESIAN_POINT('Origin',(8.,0.,1.));
#11294=CARTESIAN_POINT('',(7.5,-6.12323399573677E-17,1.));
#11295=CARTESIAN_POINT('',(7.5,-6.12323399573677E-17,1.));
#11296=CARTESIAN_POINT('Origin',(8.,0.,1.));
#11297=CARTESIAN_POINT('Origin',(8.,0.,1.));
#11854=UNCERTAINTY_MEASURE_WITH_UNIT(LENGTH_MEASURE(0.001),#11917,
'DISTANCE_ACCURACY_VALUE',
'Maximum model space distance between geometric entities at asserted c
onnectivities');
#11869=UNCERTAINTY_MEASURE_WITH_UNIT(LENGTH_MEASURE(0.001),#11917,
'DISTANCE_ACCURACY_VALUE',
'Maximum model space distance between geometric entities at asserted c
onnectivities');
#11901=(
GEOMETRIC_REPRESENTATION_CONTEXT(3)
GLOBAL_UNCERTAINTY_ASSIGNED_CONTEXT((#11854))
GLOBAL_UNIT_ASSIGNED_CONTEXT((#11917,#11919,#11920))
REPRESENTATION_CONTEXT('','3D')
);
#11916=(
GEOMETRIC_REPRESENTATION_CONTEXT(3)
GLOBAL_UNCERTAINTY_ASSIGNED_CONTEXT((#11869))
GLOBAL_UNIT_ASSIGNED_CONTEXT((#11917,#11919,#11920))
REPRESENTATION_CONTEXT('','3D')
);
#11917=(
LENGTH_UNIT()
NAMED_UNIT(*)
SI_UNIT(.CENTI.,.METRE.)
);
#11919=(
NAMED_UNIT(*)
PLANE_ANGLE_UNIT()
SI_UNIT($,.RADIAN.)
);
#11920=(
NAMED_UNIT(*)
SI_UNIT($,.STERADIAN.)
SOLID_ANGLE_UNIT()
);
#11952=SHAPE_DEFINITION_REPRESENTATION(#12003,#12110);
#12003=PRODUCT_DEFINITION_SHAPE('',$,#12157);
#12110=SHAPE_REPRESENTATION('',(#7125),#11901);
#12125=PRODUCT_DEFINITION_CONTEXT('part definition',#12265,'design');
#12157=PRODUCT_DEFINITION('Output rocker and post',
'Output rocker and post',#12203,#12125);
#12203=PRODUCT_DEFINITION_FORMATION('',$,#12298);
#12265=APPLICATION_CONTEXT(
'Core Data for Automotive Mechanical Design Process');
#12266=PRODUCT_CONTEXT('part definition',#12265,'mechanical');
#12298=PRODUCT('Output rocker and post','Output rocker and post',
'Output rocker and post',(#12266));
#12355=COLOUR_RGB('Light Blue',0.38,0.62,0.78);
#12356=FILL_AREA_STYLE_COLOUR('',#12355);
#12357=FILL_AREA_STYLE('',(#12356));
#12358=SURFACE_STYLE_FILL_AREA(#12357);
#12359=SURFACE_SIDE_STYLE('',(#12358));
#12360=SURFACE_STYLE_USAGE(.BOTH.,#12359);
#12361=PRESENTATION_STYLE_ASSIGNMENT((#12360));
ENDSEC;
END-ISO-10303-21;
